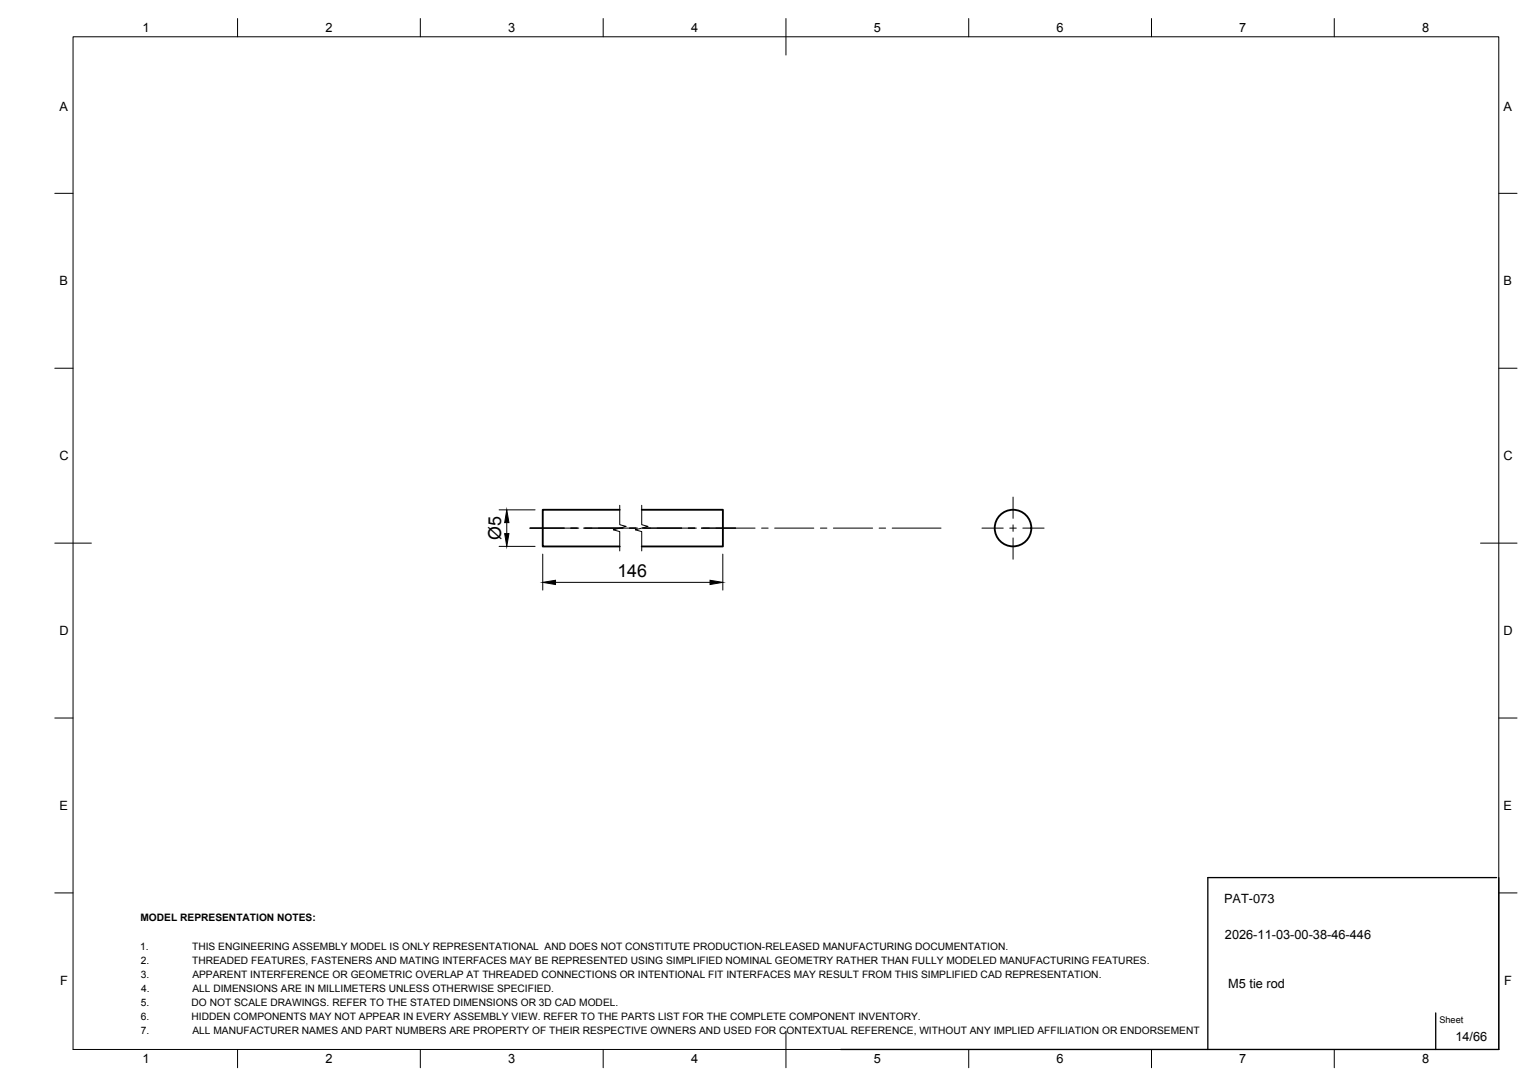
ISO-10303-21;
HEADER;
/* Generated by software containing ST-Developer
 * from STEP Tools, Inc. (www.steptools.com) 
 */

FILE_DESCRIPTION(
/* description */ ('Manual piston pump'),
/* implementation_level */ '2;1');

FILE_NAME(
/* name */ 'M5 tie rod.step',
/* time_stamp */ '2026-11-02T16:54:23-08:00',
/* author */ (''),
/* organization */ (''),
/* preprocessor_version */ 'ST-DEVELOPER v20.2',
/* originating_system */ 'Autodesk Translation Framework v15.17.0.0',
/* authorisation */ '');

FILE_SCHEMA (('AUTOMOTIVE_DESIGN { 1 0 10303 214 3 1 1 }'));
ENDSEC;

DATA;
#10=MECHANICAL_DESIGN_GEOMETRIC_PRESENTATION_REPRESENTATION('',(#697),#19043);
#571=SHAPE_REPRESENTATION_RELATIONSHIP('SRR','None',#19317,#634);
#634=ADVANCED_BREP_SHAPE_REPRESENTATION('',(#769),#18984);
#697=STYLED_ITEM('',(#19661),#769);
#769=MANIFOLD_SOLID_BREP('Body1',#9481);
#1138=CYLINDRICAL_SURFACE('',#10454,0.25);
#1393=FACE_OUTER_BOUND('',#2025,.T.);
#1394=FACE_OUTER_BOUND('',#2026,.T.);
#1395=FACE_OUTER_BOUND('',#2027,.T.);
#2025=EDGE_LOOP('',(#6711,#6712,#6713,#6714));
#2026=EDGE_LOOP('',(#6715));
#2027=EDGE_LOOP('',(#6716));
#2761=CIRCLE('',#10455,0.25);
#2762=CIRCLE('',#10456,0.25);
#3265=LINE('',#15135,#3869);
#3869=VECTOR('',#12039,0.25);
#4500=VERTEX_POINT('',#15132);
#4501=VERTEX_POINT('',#15134);
#5342=EDGE_CURVE('',#4500,#4500,#2761,.T.);
#5343=EDGE_CURVE('',#4500,#4501,#3265,.T.);
#5344=EDGE_CURVE('',#4501,#4501,#2762,.T.);
#6711=ORIENTED_EDGE('',*,*,#5342,.F.);
#6712=ORIENTED_EDGE('',*,*,#5343,.T.);
#6713=ORIENTED_EDGE('',*,*,#5344,.T.);
#6714=ORIENTED_EDGE('',*,*,#5343,.F.);
#6715=ORIENTED_EDGE('',*,*,#5342,.T.);
#6716=ORIENTED_EDGE('',*,*,#5344,.F.);
#8626=PLANE('',#10457);
#8627=PLANE('',#10458);
#8998=ADVANCED_FACE('',(#1393),#1138,.T.);
#8999=ADVANCED_FACE('',(#1394),#8626,.T.);
#9000=ADVANCED_FACE('',(#1395),#8627,.F.);
#9481=CLOSED_SHELL('',(#8998,#8999,#9000));
#10453=AXIS2_PLACEMENT_3D('',#15130,#12033,#12034);
#10454=AXIS2_PLACEMENT_3D('',#15131,#12035,#12036);
#10455=AXIS2_PLACEMENT_3D('',#15133,#12037,#12038);
#10456=AXIS2_PLACEMENT_3D('',#15136,#12040,#12041);
#10457=AXIS2_PLACEMENT_3D('',#15137,#12042,#12043);
#10458=AXIS2_PLACEMENT_3D('',#15138,#12044,#12045);
#12033=DIRECTION('axis',(0.,0.,1.));
#12034=DIRECTION('refdir',(1.,0.,0.));
#12035=DIRECTION('center_axis',(0.,1.,0.));
#12036=DIRECTION('ref_axis',(1.,0.,0.));
#12037=DIRECTION('center_axis',(0.,1.,0.));
#12038=DIRECTION('ref_axis',(1.,0.,0.));
#12039=DIRECTION('',(0.,-1.,0.));
#12040=DIRECTION('center_axis',(0.,1.,0.));
#12041=DIRECTION('ref_axis',(1.,0.,0.));
#12042=DIRECTION('center_axis',(0.,1.,0.));
#12043=DIRECTION('ref_axis',(1.,0.,0.));
#12044=DIRECTION('center_axis',(0.,1.,0.));
#12045=DIRECTION('ref_axis',(1.,0.,0.));
#15130=CARTESIAN_POINT('',(0.,0.,0.));
#15131=CARTESIAN_POINT('Origin',(-2.,-1.,2.5));
#15132=CARTESIAN_POINT('',(-2.25,13.6,2.5));
#15133=CARTESIAN_POINT('Origin',(-2.,13.6,2.5));
#15134=CARTESIAN_POINT('',(-2.25,-1.,2.5));
#15135=CARTESIAN_POINT('',(-2.25,-1.,2.5));
#15136=CARTESIAN_POINT('Origin',(-2.,-1.,2.5));
#15137=CARTESIAN_POINT('Origin',(-2.,13.6,2.5));
#15138=CARTESIAN_POINT('Origin',(-2.,-1.,2.5));
#18913=UNCERTAINTY_MEASURE_WITH_UNIT(LENGTH_MEASURE(0.001),#19044,
'DISTANCE_ACCURACY_VALUE',
'Maximum model space distance between geometric entities at asserted c
onnectivities');
#18972=UNCERTAINTY_MEASURE_WITH_UNIT(LENGTH_MEASURE(0.001),#19044,
'DISTANCE_ACCURACY_VALUE',
'Maximum model space distance between geometric entities at asserted c
onnectivities');
#18984=(
GEOMETRIC_REPRESENTATION_CONTEXT(3)
GLOBAL_UNCERTAINTY_ASSIGNED_CONTEXT((#18913))
GLOBAL_UNIT_ASSIGNED_CONTEXT((#19044,#19046,#19047))
REPRESENTATION_CONTEXT('','3D')
);
#19043=(
GEOMETRIC_REPRESENTATION_CONTEXT(3)
GLOBAL_UNCERTAINTY_ASSIGNED_CONTEXT((#18972))
GLOBAL_UNIT_ASSIGNED_CONTEXT((#19044,#19046,#19047))
REPRESENTATION_CONTEXT('','3D')
);
#19044=(
LENGTH_UNIT()
NAMED_UNIT(*)
SI_UNIT(.CENTI.,.METRE.)
);
#19046=(
NAMED_UNIT(*)
PLANE_ANGLE_UNIT()
SI_UNIT($,.RADIAN.)
);
#19047=(
NAMED_UNIT(*)
SI_UNIT($,.STERADIAN.)
SOLID_ANGLE_UNIT()
);
#19059=SHAPE_DEFINITION_REPRESENTATION(#19129,#19317);
#19129=PRODUCT_DEFINITION_SHAPE('',$,#19388);
#19317=SHAPE_REPRESENTATION('',(#10453),#18984);
#19376=PRODUCT_DEFINITION_CONTEXT('part definition',#19588,'design');
#19388=PRODUCT_DEFINITION('2026-11-03-00-38-46-446','M5 tie rod',#19458,
#19376);
#19458=PRODUCT_DEFINITION_FORMATION('',$,#19601);
#19588=APPLICATION_CONTEXT(
'Core Data for Automotive Mechanical Design Process');
#19589=PRODUCT_CONTEXT('part definition',#19588,'mechanical');
#19601=PRODUCT('2026-11-03-00-38-46-446','M5 tie rod','M5 tie rod',(#19589));
#19661=PRESENTATION_STYLE_ASSIGNMENT((#19667));
#19667=SURFACE_STYLE_USAGE(.BOTH.,#19673);
#19673=SURFACE_SIDE_STYLE('',(#19679));
#19679=SURFACE_STYLE_FILL_AREA(#19685);
#19685=FILL_AREA_STYLE('CAD Library Painted - Engineering blue',(#19691));
#19691=FILL_AREA_STYLE_COLOUR('CAD Library Painted - Engineering blue',
#19697);
#19697=COLOUR_RGB('CAD Library Painted - Engineering blue',0.12156862745098,
0.356862745098039,0.6);
ENDSEC;
END-ISO-10303-21;
